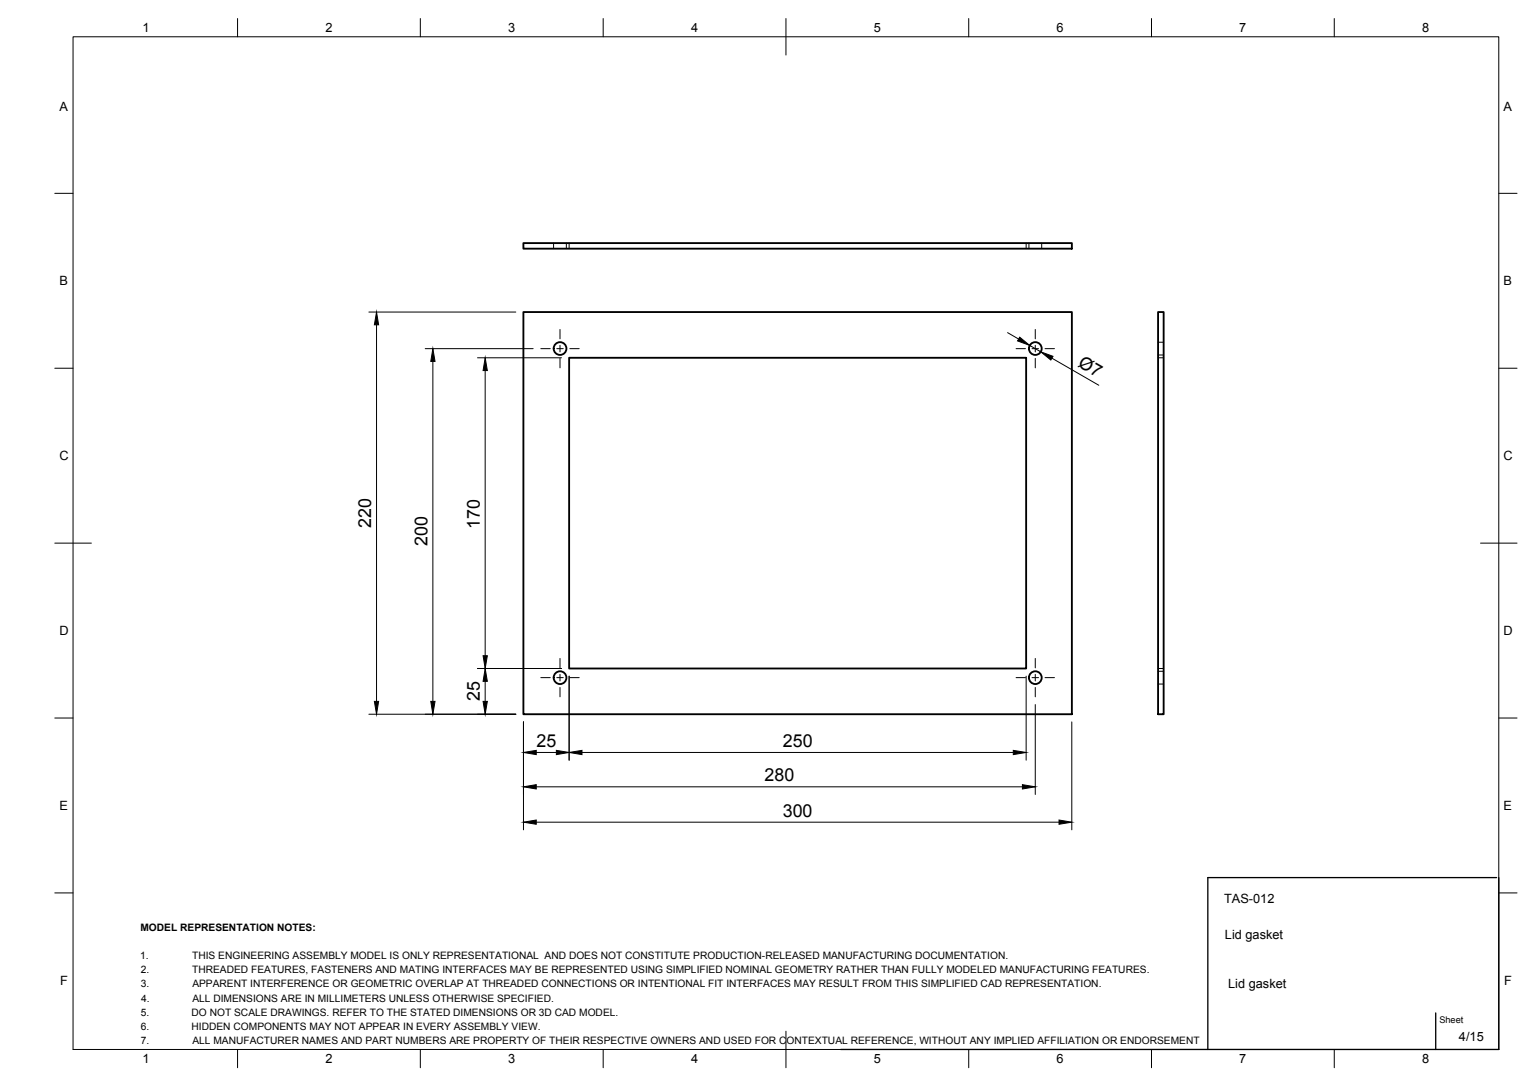
ISO-10303-21;
HEADER;
/* Generated by software containing ST-Developer
 * from STEP Tools, Inc. (www.steptools.com) 
 */

FILE_DESCRIPTION(
/* description */ (
'Independent welded steel electronics enclosure with removable sealed 
lid, internal mounting tray and two threaded cable entries. 300 x 220 
mm body. No ingress or electrical safety rating assigned.'),
/* implementation_level */ '2;1');

FILE_NAME(
/* name */ 'Lid gasket.step',
/* time_stamp */ '2026-11-14T09:13:27-08:00',
/* author */ (''),
/* organization */ (''),
/* preprocessor_version */ 'ST-DEVELOPER v20.2',
/* originating_system */ 'Autodesk Translation Framework v15.17.0.0',
/* authorisation */ '');

FILE_SCHEMA (('AUTOMOTIVE_DESIGN { 1 0 10303 214 3 1 1 }'));
ENDSEC;

DATA;
#10=MECHANICAL_DESIGN_GEOMETRIC_PRESENTATION_REPRESENTATION('',(#974),#94412);
#944=SHAPE_REPRESENTATION_RELATIONSHIP('SRR','None',#94496,#959);
#959=ADVANCED_BREP_SHAPE_REPRESENTATION('',(#989),#94405);
#974=STYLED_ITEM('',(#94578),#989);
#989=MANIFOLD_SOLID_BREP('Body1',#8259);
#1025=FACE_BOUND('',#1770,.T.);
#1026=FACE_BOUND('',#1771,.T.);
#1027=FACE_BOUND('',#1772,.T.);
#1028=FACE_BOUND('',#1773,.T.);
#1029=FACE_BOUND('',#1774,.T.);
#1030=FACE_BOUND('',#1776,.T.);
#1031=FACE_BOUND('',#1777,.T.);
#1032=FACE_BOUND('',#1778,.T.);
#1033=FACE_BOUND('',#1779,.T.);
#1034=FACE_BOUND('',#1780,.T.);
#1115=PLANE('',#8744);
#1116=PLANE('',#8745);
#1117=PLANE('',#8746);
#1118=PLANE('',#8747);
#1119=PLANE('',#8748);
#1120=PLANE('',#8749);
#1121=PLANE('',#8750);
#1122=PLANE('',#8751);
#1123=PLANE('',#8752);
#1124=PLANE('',#8753);
#1372=FACE_OUTER_BOUND('',#1757,.T.);
#1373=FACE_OUTER_BOUND('',#1758,.T.);
#1374=FACE_OUTER_BOUND('',#1759,.T.);
#1375=FACE_OUTER_BOUND('',#1760,.T.);
#1376=FACE_OUTER_BOUND('',#1761,.T.);
#1377=FACE_OUTER_BOUND('',#1762,.T.);
#1378=FACE_OUTER_BOUND('',#1763,.T.);
#1379=FACE_OUTER_BOUND('',#1764,.T.);
#1380=FACE_OUTER_BOUND('',#1765,.T.);
#1381=FACE_OUTER_BOUND('',#1766,.T.);
#1382=FACE_OUTER_BOUND('',#1767,.T.);
#1383=FACE_OUTER_BOUND('',#1768,.T.);
#1384=FACE_OUTER_BOUND('',#1769,.T.);
#1385=FACE_OUTER_BOUND('',#1775,.T.);
#1757=EDGE_LOOP('',(#6692,#6693,#6694,#6695));
#1758=EDGE_LOOP('',(#6696,#6697,#6698,#6699));
#1759=EDGE_LOOP('',(#6700,#6701,#6702,#6703));
#1760=EDGE_LOOP('',(#6704,#6705,#6706,#6707));
#1761=EDGE_LOOP('',(#6708,#6709,#6710,#6711));
#1762=EDGE_LOOP('',(#6712,#6713,#6714,#6715));
#1763=EDGE_LOOP('',(#6716,#6717,#6718,#6719));
#1764=EDGE_LOOP('',(#6720,#6721,#6722,#6723));
#1765=EDGE_LOOP('',(#6724,#6725,#6726,#6727));
#1766=EDGE_LOOP('',(#6728,#6729,#6730,#6731));
#1767=EDGE_LOOP('',(#6732,#6733,#6734,#6735));
#1768=EDGE_LOOP('',(#6736,#6737,#6738,#6739));
#1769=EDGE_LOOP('',(#6740,#6741,#6742,#6743));
#1770=EDGE_LOOP('',(#6744,#6745,#6746,#6747));
#1771=EDGE_LOOP('',(#6748));
#1772=EDGE_LOOP('',(#6749));
#1773=EDGE_LOOP('',(#6750));
#1774=EDGE_LOOP('',(#6751));
#1775=EDGE_LOOP('',(#6752,#6753,#6754,#6755));
#1776=EDGE_LOOP('',(#6756,#6757,#6758,#6759));
#1777=EDGE_LOOP('',(#6760));
#1778=EDGE_LOOP('',(#6761));
#1779=EDGE_LOOP('',(#6762));
#1780=EDGE_LOOP('',(#6763));
#2175=LINE('',#59753,#2573);
#2176=LINE('',#59759,#2574);
#2177=LINE('',#59765,#2575);
#2178=LINE('',#59771,#2576);
#2179=LINE('',#59776,#2577);
#2180=LINE('',#59778,#2578);
#2181=LINE('',#59780,#2579);
#2182=LINE('',#59781,#2580);
#2183=LINE('',#59784,#2581);
#2184=LINE('',#59786,#2582);
#2185=LINE('',#59787,#2583);
#2186=LINE('',#59790,#2584);
#2187=LINE('',#59792,#2585);
#2188=LINE('',#59793,#2586);
#2189=LINE('',#59795,#2587);
#2190=LINE('',#59796,#2588);
#2191=LINE('',#59800,#2589);
#2192=LINE('',#59802,#2590);
#2193=LINE('',#59804,#2591);
#2194=LINE('',#59805,#2592);
#2195=LINE('',#59808,#2593);
#2196=LINE('',#59810,#2594);
#2197=LINE('',#59811,#2595);
#2198=LINE('',#59814,#2596);
#2199=LINE('',#59816,#2597);
#2200=LINE('',#59817,#2598);
#2201=LINE('',#59819,#2599);
#2202=LINE('',#59820,#2600);
#2573=VECTOR('',#9789,3.5);
#2574=VECTOR('',#9796,3.5);
#2575=VECTOR('',#9803,3.5);
#2576=VECTOR('',#9810,3.5);
#2577=VECTOR('',#9815,10.);
#2578=VECTOR('',#9816,10.);
#2579=VECTOR('',#9817,10.);
#2580=VECTOR('',#9818,10.);
#2581=VECTOR('',#9821,10.);
#2582=VECTOR('',#9822,10.);
#2583=VECTOR('',#9823,10.);
#2584=VECTOR('',#9826,10.);
#2585=VECTOR('',#9827,10.);
#2586=VECTOR('',#9828,10.);
#2587=VECTOR('',#9831,10.);
#2588=VECTOR('',#9832,10.);
#2589=VECTOR('',#9835,10.);
#2590=VECTOR('',#9836,10.);
#2591=VECTOR('',#9837,10.);
#2592=VECTOR('',#9838,10.);
#2593=VECTOR('',#9841,10.);
#2594=VECTOR('',#9842,10.);
#2595=VECTOR('',#9843,10.);
#2596=VECTOR('',#9846,10.);
#2597=VECTOR('',#9847,10.);
#2598=VECTOR('',#9848,10.);
#2599=VECTOR('',#9851,10.);
#2600=VECTOR('',#9852,10.);
#2794=CIRCLE('',#8733,3.5);
#2795=CIRCLE('',#8734,3.5);
#2796=CIRCLE('',#8736,3.5);
#2797=CIRCLE('',#8737,3.5);
#2798=CIRCLE('',#8739,3.5);
#2799=CIRCLE('',#8740,3.5);
#2800=CIRCLE('',#8742,3.5);
#2801=CIRCLE('',#8743,3.5);
#3452=VERTEX_POINT('',#59750);
#3453=VERTEX_POINT('',#59752);
#3454=VERTEX_POINT('',#59756);
#3455=VERTEX_POINT('',#59758);
#3456=VERTEX_POINT('',#59762);
#3457=VERTEX_POINT('',#59764);
#3458=VERTEX_POINT('',#59768);
#3459=VERTEX_POINT('',#59770);
#3460=VERTEX_POINT('',#59774);
#3461=VERTEX_POINT('',#59775);
#3462=VERTEX_POINT('',#59777);
#3463=VERTEX_POINT('',#59779);
#3464=VERTEX_POINT('',#59783);
#3465=VERTEX_POINT('',#59785);
#3466=VERTEX_POINT('',#59789);
#3467=VERTEX_POINT('',#59791);
#3468=VERTEX_POINT('',#59798);
#3469=VERTEX_POINT('',#59799);
#3470=VERTEX_POINT('',#59801);
#3471=VERTEX_POINT('',#59803);
#3472=VERTEX_POINT('',#59807);
#3473=VERTEX_POINT('',#59809);
#3474=VERTEX_POINT('',#59813);
#3475=VERTEX_POINT('',#59815);
#4611=EDGE_CURVE('',#3452,#3452,#2794,.T.);
#4612=EDGE_CURVE('',#3452,#3453,#2175,.T.);
#4613=EDGE_CURVE('',#3453,#3453,#2795,.T.);
#4614=EDGE_CURVE('',#3454,#3454,#2796,.T.);
#4615=EDGE_CURVE('',#3454,#3455,#2176,.T.);
#4616=EDGE_CURVE('',#3455,#3455,#2797,.T.);
#4617=EDGE_CURVE('',#3456,#3456,#2798,.T.);
#4618=EDGE_CURVE('',#3456,#3457,#2177,.T.);
#4619=EDGE_CURVE('',#3457,#3457,#2799,.T.);
#4620=EDGE_CURVE('',#3458,#3458,#2800,.T.);
#4621=EDGE_CURVE('',#3458,#3459,#2178,.T.);
#4622=EDGE_CURVE('',#3459,#3459,#2801,.T.);
#4623=EDGE_CURVE('',#3460,#3461,#2179,.T.);
#4624=EDGE_CURVE('',#3461,#3462,#2180,.T.);
#4625=EDGE_CURVE('',#3463,#3462,#2181,.T.);
#4626=EDGE_CURVE('',#3460,#3463,#2182,.T.);
#4627=EDGE_CURVE('',#3464,#3460,#2183,.T.);
#4628=EDGE_CURVE('',#3465,#3463,#2184,.T.);
#4629=EDGE_CURVE('',#3464,#3465,#2185,.T.);
#4630=EDGE_CURVE('',#3466,#3464,#2186,.T.);
#4631=EDGE_CURVE('',#3467,#3465,#2187,.T.);
#4632=EDGE_CURVE('',#3466,#3467,#2188,.T.);
#4633=EDGE_CURVE('',#3461,#3466,#2189,.T.);
#4634=EDGE_CURVE('',#3462,#3467,#2190,.T.);
#4635=EDGE_CURVE('',#3468,#3469,#2191,.T.);
#4636=EDGE_CURVE('',#3469,#3470,#2192,.T.);
#4637=EDGE_CURVE('',#3471,#3470,#2193,.T.);
#4638=EDGE_CURVE('',#3468,#3471,#2194,.T.);
#4639=EDGE_CURVE('',#3472,#3468,#2195,.T.);
#4640=EDGE_CURVE('',#3473,#3471,#2196,.T.);
#4641=EDGE_CURVE('',#3472,#3473,#2197,.T.);
#4642=EDGE_CURVE('',#3474,#3472,#2198,.T.);
#4643=EDGE_CURVE('',#3475,#3473,#2199,.T.);
#4644=EDGE_CURVE('',#3474,#3475,#2200,.T.);
#4645=EDGE_CURVE('',#3469,#3474,#2201,.T.);
#4646=EDGE_CURVE('',#3470,#3475,#2202,.T.);
#6692=ORIENTED_EDGE('',*,*,#4611,.F.);
#6693=ORIENTED_EDGE('',*,*,#4612,.T.);
#6694=ORIENTED_EDGE('',*,*,#4613,.F.);
#6695=ORIENTED_EDGE('',*,*,#4612,.F.);
#6696=ORIENTED_EDGE('',*,*,#4614,.F.);
#6697=ORIENTED_EDGE('',*,*,#4615,.T.);
#6698=ORIENTED_EDGE('',*,*,#4616,.F.);
#6699=ORIENTED_EDGE('',*,*,#4615,.F.);
#6700=ORIENTED_EDGE('',*,*,#4617,.F.);
#6701=ORIENTED_EDGE('',*,*,#4618,.T.);
#6702=ORIENTED_EDGE('',*,*,#4619,.F.);
#6703=ORIENTED_EDGE('',*,*,#4618,.F.);
#6704=ORIENTED_EDGE('',*,*,#4620,.F.);
#6705=ORIENTED_EDGE('',*,*,#4621,.T.);
#6706=ORIENTED_EDGE('',*,*,#4622,.F.);
#6707=ORIENTED_EDGE('',*,*,#4621,.F.);
#6708=ORIENTED_EDGE('',*,*,#4623,.T.);
#6709=ORIENTED_EDGE('',*,*,#4624,.T.);
#6710=ORIENTED_EDGE('',*,*,#4625,.F.);
#6711=ORIENTED_EDGE('',*,*,#4626,.F.);
#6712=ORIENTED_EDGE('',*,*,#4627,.T.);
#6713=ORIENTED_EDGE('',*,*,#4626,.T.);
#6714=ORIENTED_EDGE('',*,*,#4628,.F.);
#6715=ORIENTED_EDGE('',*,*,#4629,.F.);
#6716=ORIENTED_EDGE('',*,*,#4630,.T.);
#6717=ORIENTED_EDGE('',*,*,#4629,.T.);
#6718=ORIENTED_EDGE('',*,*,#4631,.F.);
#6719=ORIENTED_EDGE('',*,*,#4632,.F.);
#6720=ORIENTED_EDGE('',*,*,#4633,.T.);
#6721=ORIENTED_EDGE('',*,*,#4632,.T.);
#6722=ORIENTED_EDGE('',*,*,#4634,.F.);
#6723=ORIENTED_EDGE('',*,*,#4624,.F.);
#6724=ORIENTED_EDGE('',*,*,#4635,.T.);
#6725=ORIENTED_EDGE('',*,*,#4636,.T.);
#6726=ORIENTED_EDGE('',*,*,#4637,.F.);
#6727=ORIENTED_EDGE('',*,*,#4638,.F.);
#6728=ORIENTED_EDGE('',*,*,#4639,.T.);
#6729=ORIENTED_EDGE('',*,*,#4638,.T.);
#6730=ORIENTED_EDGE('',*,*,#4640,.F.);
#6731=ORIENTED_EDGE('',*,*,#4641,.F.);
#6732=ORIENTED_EDGE('',*,*,#4642,.T.);
#6733=ORIENTED_EDGE('',*,*,#4641,.T.);
#6734=ORIENTED_EDGE('',*,*,#4643,.F.);
#6735=ORIENTED_EDGE('',*,*,#4644,.F.);
#6736=ORIENTED_EDGE('',*,*,#4645,.T.);
#6737=ORIENTED_EDGE('',*,*,#4644,.T.);
#6738=ORIENTED_EDGE('',*,*,#4646,.F.);
#6739=ORIENTED_EDGE('',*,*,#4636,.F.);
#6740=ORIENTED_EDGE('',*,*,#4646,.T.);
#6741=ORIENTED_EDGE('',*,*,#4643,.T.);
#6742=ORIENTED_EDGE('',*,*,#4640,.T.);
#6743=ORIENTED_EDGE('',*,*,#4637,.T.);
#6744=ORIENTED_EDGE('',*,*,#4634,.T.);
#6745=ORIENTED_EDGE('',*,*,#4631,.T.);
#6746=ORIENTED_EDGE('',*,*,#4628,.T.);
#6747=ORIENTED_EDGE('',*,*,#4625,.T.);
#6748=ORIENTED_EDGE('',*,*,#4620,.T.);
#6749=ORIENTED_EDGE('',*,*,#4617,.T.);
#6750=ORIENTED_EDGE('',*,*,#4614,.T.);
#6751=ORIENTED_EDGE('',*,*,#4611,.T.);
#6752=ORIENTED_EDGE('',*,*,#4645,.F.);
#6753=ORIENTED_EDGE('',*,*,#4635,.F.);
#6754=ORIENTED_EDGE('',*,*,#4639,.F.);
#6755=ORIENTED_EDGE('',*,*,#4642,.F.);
#6756=ORIENTED_EDGE('',*,*,#4633,.F.);
#6757=ORIENTED_EDGE('',*,*,#4623,.F.);
#6758=ORIENTED_EDGE('',*,*,#4627,.F.);
#6759=ORIENTED_EDGE('',*,*,#4630,.F.);
#6760=ORIENTED_EDGE('',*,*,#4622,.T.);
#6761=ORIENTED_EDGE('',*,*,#4619,.T.);
#6762=ORIENTED_EDGE('',*,*,#4616,.T.);
#6763=ORIENTED_EDGE('',*,*,#4613,.T.);
#7806=CYLINDRICAL_SURFACE('',#8732,3.5);
#7807=CYLINDRICAL_SURFACE('',#8735,3.5);
#7808=CYLINDRICAL_SURFACE('',#8738,3.5);
#7809=CYLINDRICAL_SURFACE('',#8741,3.5);
#8109=ADVANCED_FACE('',(#1372),#7806,.F.);
#8110=ADVANCED_FACE('',(#1373),#7807,.F.);
#8111=ADVANCED_FACE('',(#1374),#7808,.F.);
#8112=ADVANCED_FACE('',(#1375),#7809,.F.);
#8113=ADVANCED_FACE('',(#1376),#1115,.T.);
#8114=ADVANCED_FACE('',(#1377),#1116,.T.);
#8115=ADVANCED_FACE('',(#1378),#1117,.T.);
#8116=ADVANCED_FACE('',(#1379),#1118,.T.);
#8117=ADVANCED_FACE('',(#1380),#1119,.T.);
#8118=ADVANCED_FACE('',(#1381),#1120,.T.);
#8119=ADVANCED_FACE('',(#1382),#1121,.T.);
#8120=ADVANCED_FACE('',(#1383),#1122,.T.);
#8121=ADVANCED_FACE('',(#1384,#1025,#1026,#1027,#1028,#1029),#1123,.T.);
#8122=ADVANCED_FACE('',(#1385,#1030,#1031,#1032,#1033,#1034),#1124,.F.);
#8259=CLOSED_SHELL('',(#8109,#8110,#8111,#8112,#8113,#8114,#8115,#8116,
#8117,#8118,#8119,#8120,#8121,#8122));
#8731=AXIS2_PLACEMENT_3D('',#59748,#9783,#9784);
#8732=AXIS2_PLACEMENT_3D('',#59749,#9785,#9786);
#8733=AXIS2_PLACEMENT_3D('',#59751,#9787,#9788);
#8734=AXIS2_PLACEMENT_3D('',#59754,#9790,#9791);
#8735=AXIS2_PLACEMENT_3D('',#59755,#9792,#9793);
#8736=AXIS2_PLACEMENT_3D('',#59757,#9794,#9795);
#8737=AXIS2_PLACEMENT_3D('',#59760,#9797,#9798);
#8738=AXIS2_PLACEMENT_3D('',#59761,#9799,#9800);
#8739=AXIS2_PLACEMENT_3D('',#59763,#9801,#9802);
#8740=AXIS2_PLACEMENT_3D('',#59766,#9804,#9805);
#8741=AXIS2_PLACEMENT_3D('',#59767,#9806,#9807);
#8742=AXIS2_PLACEMENT_3D('',#59769,#9808,#9809);
#8743=AXIS2_PLACEMENT_3D('',#59772,#9811,#9812);
#8744=AXIS2_PLACEMENT_3D('',#59773,#9813,#9814);
#8745=AXIS2_PLACEMENT_3D('',#59782,#9819,#9820);
#8746=AXIS2_PLACEMENT_3D('',#59788,#9824,#9825);
#8747=AXIS2_PLACEMENT_3D('',#59794,#9829,#9830);
#8748=AXIS2_PLACEMENT_3D('',#59797,#9833,#9834);
#8749=AXIS2_PLACEMENT_3D('',#59806,#9839,#9840);
#8750=AXIS2_PLACEMENT_3D('',#59812,#9844,#9845);
#8751=AXIS2_PLACEMENT_3D('',#59818,#9849,#9850);
#8752=AXIS2_PLACEMENT_3D('',#59821,#9853,#9854);
#8753=AXIS2_PLACEMENT_3D('',#59822,#9855,#9856);
#9783=DIRECTION('axis',(0.,0.,1.));
#9784=DIRECTION('refdir',(1.,0.,0.));
#9785=DIRECTION('center_axis',(0.,0.,-1.));
#9786=DIRECTION('ref_axis',(1.,0.,0.));
#9787=DIRECTION('center_axis',(0.,0.,-1.));
#9788=DIRECTION('ref_axis',(1.,0.,0.));
#9789=DIRECTION('',(0.,0.,-1.));
#9790=DIRECTION('center_axis',(0.,0.,1.));
#9791=DIRECTION('ref_axis',(1.,0.,0.));
#9792=DIRECTION('center_axis',(0.,0.,-1.));
#9793=DIRECTION('ref_axis',(1.,0.,0.));
#9794=DIRECTION('center_axis',(0.,0.,-1.));
#9795=DIRECTION('ref_axis',(1.,0.,0.));
#9796=DIRECTION('',(0.,0.,-1.));
#9797=DIRECTION('center_axis',(0.,0.,1.));
#9798=DIRECTION('ref_axis',(1.,0.,0.));
#9799=DIRECTION('center_axis',(0.,0.,-1.));
#9800=DIRECTION('ref_axis',(1.,0.,0.));
#9801=DIRECTION('center_axis',(0.,0.,-1.));
#9802=DIRECTION('ref_axis',(1.,0.,0.));
#9803=DIRECTION('',(0.,0.,-1.));
#9804=DIRECTION('center_axis',(0.,0.,1.));
#9805=DIRECTION('ref_axis',(1.,0.,0.));
#9806=DIRECTION('center_axis',(0.,0.,-1.));
#9807=DIRECTION('ref_axis',(1.,0.,0.));
#9808=DIRECTION('center_axis',(0.,0.,-1.));
#9809=DIRECTION('ref_axis',(1.,0.,0.));
#9810=DIRECTION('',(0.,0.,-1.));
#9811=DIRECTION('center_axis',(0.,0.,1.));
#9812=DIRECTION('ref_axis',(1.,0.,0.));
#9813=DIRECTION('center_axis',(0.,1.,0.));
#9814=DIRECTION('ref_axis',(-1.,0.,0.));
#9815=DIRECTION('',(-1.,0.,0.));
#9816=DIRECTION('',(0.,0.,1.));
#9817=DIRECTION('',(-1.,0.,0.));
#9818=DIRECTION('',(0.,0.,1.));
#9819=DIRECTION('center_axis',(-1.,0.,0.));
#9820=DIRECTION('ref_axis',(0.,-1.,0.));
#9821=DIRECTION('',(0.,-1.,0.));
#9822=DIRECTION('',(0.,-1.,0.));
#9823=DIRECTION('',(0.,0.,1.));
#9824=DIRECTION('center_axis',(0.,-1.,0.));
#9825=DIRECTION('ref_axis',(1.,0.,0.));
#9826=DIRECTION('',(1.,0.,0.));
#9827=DIRECTION('',(1.,0.,0.));
#9828=DIRECTION('',(0.,0.,1.));
#9829=DIRECTION('center_axis',(1.,0.,0.));
#9830=DIRECTION('ref_axis',(0.,1.,0.));
#9831=DIRECTION('',(0.,1.,0.));
#9832=DIRECTION('',(0.,1.,0.));
#9833=DIRECTION('center_axis',(0.,1.,0.));
#9834=DIRECTION('ref_axis',(-1.,0.,0.));
#9835=DIRECTION('',(-1.,0.,0.));
#9836=DIRECTION('',(0.,0.,1.));
#9837=DIRECTION('',(-1.,0.,0.));
#9838=DIRECTION('',(0.,0.,1.));
#9839=DIRECTION('center_axis',(1.,0.,0.));
#9840=DIRECTION('ref_axis',(0.,1.,0.));
#9841=DIRECTION('',(0.,1.,0.));
#9842=DIRECTION('',(0.,1.,0.));
#9843=DIRECTION('',(0.,0.,1.));
#9844=DIRECTION('center_axis',(0.,-1.,0.));
#9845=DIRECTION('ref_axis',(1.,0.,0.));
#9846=DIRECTION('',(1.,0.,0.));
#9847=DIRECTION('',(1.,0.,0.));
#9848=DIRECTION('',(0.,0.,1.));
#9849=DIRECTION('center_axis',(-1.,0.,0.));
#9850=DIRECTION('ref_axis',(0.,-1.,0.));
#9851=DIRECTION('',(0.,-1.,0.));
#9852=DIRECTION('',(0.,-1.,0.));
#9853=DIRECTION('center_axis',(0.,0.,1.));
#9854=DIRECTION('ref_axis',(1.,0.,0.));
#9855=DIRECTION('center_axis',(0.,0.,1.));
#9856=DIRECTION('ref_axis',(1.,0.,0.));
#59748=CARTESIAN_POINT('',(0.,0.,0.));
#59749=CARTESIAN_POINT('Origin',(130.,-90.,1.5));
#59750=CARTESIAN_POINT('',(126.5,-90.,3.));
#59751=CARTESIAN_POINT('Origin',(130.,-90.,3.));
#59752=CARTESIAN_POINT('',(126.5,-90.,0.));
#59753=CARTESIAN_POINT('',(126.5,-90.,1.5));
#59754=CARTESIAN_POINT('Origin',(130.,-90.,0.));
#59755=CARTESIAN_POINT('Origin',(-130.,-90.,1.5));
#59756=CARTESIAN_POINT('',(-133.5,-90.,3.));
#59757=CARTESIAN_POINT('Origin',(-130.,-90.,3.));
#59758=CARTESIAN_POINT('',(-133.5,-90.,0.));
#59759=CARTESIAN_POINT('',(-133.5,-90.,1.5));
#59760=CARTESIAN_POINT('Origin',(-130.,-90.,0.));
#59761=CARTESIAN_POINT('Origin',(-130.,90.,1.5));
#59762=CARTESIAN_POINT('',(-133.5,90.,3.));
#59763=CARTESIAN_POINT('Origin',(-130.,90.,3.));
#59764=CARTESIAN_POINT('',(-133.5,90.,0.));
#59765=CARTESIAN_POINT('',(-133.5,90.,1.5));
#59766=CARTESIAN_POINT('Origin',(-130.,90.,0.));
#59767=CARTESIAN_POINT('Origin',(130.,90.,1.5));
#59768=CARTESIAN_POINT('',(126.5,90.,3.));
#59769=CARTESIAN_POINT('Origin',(130.,90.,3.));
#59770=CARTESIAN_POINT('',(126.5,90.,0.));
#59771=CARTESIAN_POINT('',(126.5,90.,1.5));
#59772=CARTESIAN_POINT('Origin',(130.,90.,0.));
#59773=CARTESIAN_POINT('Origin',(125.,-85.,0.));
#59774=CARTESIAN_POINT('',(125.,-85.,0.));
#59775=CARTESIAN_POINT('',(-125.,-85.,0.));
#59776=CARTESIAN_POINT('',(-125.,-85.,0.));
#59777=CARTESIAN_POINT('',(-125.,-85.,3.));
#59778=CARTESIAN_POINT('',(-125.,-85.,0.));
#59779=CARTESIAN_POINT('',(125.,-85.,3.));
#59780=CARTESIAN_POINT('',(-125.,-85.,3.));
#59781=CARTESIAN_POINT('',(125.,-85.,0.));
#59782=CARTESIAN_POINT('Origin',(125.,85.,0.));
#59783=CARTESIAN_POINT('',(125.,85.,0.));
#59784=CARTESIAN_POINT('',(125.,-85.,0.));
#59785=CARTESIAN_POINT('',(125.,85.,3.));
#59786=CARTESIAN_POINT('',(125.,-85.,3.));
#59787=CARTESIAN_POINT('',(125.,85.,0.));
#59788=CARTESIAN_POINT('Origin',(-125.,85.,0.));
#59789=CARTESIAN_POINT('',(-125.,85.,0.));
#59790=CARTESIAN_POINT('',(125.,85.,0.));
#59791=CARTESIAN_POINT('',(-125.,85.,3.));
#59792=CARTESIAN_POINT('',(125.,85.,3.));
#59793=CARTESIAN_POINT('',(-125.,85.,0.));
#59794=CARTESIAN_POINT('Origin',(-125.,-85.,0.));
#59795=CARTESIAN_POINT('',(-125.,85.,0.));
#59796=CARTESIAN_POINT('',(-125.,85.,3.));
#59797=CARTESIAN_POINT('Origin',(150.,110.,0.));
#59798=CARTESIAN_POINT('',(150.,110.,0.));
#59799=CARTESIAN_POINT('',(-150.,110.,0.));
#59800=CARTESIAN_POINT('',(150.,110.,0.));
#59801=CARTESIAN_POINT('',(-150.,110.,3.));
#59802=CARTESIAN_POINT('',(-150.,110.,0.));
#59803=CARTESIAN_POINT('',(150.,110.,3.));
#59804=CARTESIAN_POINT('',(150.,110.,3.));
#59805=CARTESIAN_POINT('',(150.,110.,0.));
#59806=CARTESIAN_POINT('Origin',(150.,-110.,0.));
#59807=CARTESIAN_POINT('',(150.,-110.,0.));
#59808=CARTESIAN_POINT('',(150.,-110.,0.));
#59809=CARTESIAN_POINT('',(150.,-110.,3.));
#59810=CARTESIAN_POINT('',(150.,-110.,3.));
#59811=CARTESIAN_POINT('',(150.,-110.,0.));
#59812=CARTESIAN_POINT('Origin',(-150.,-110.,0.));
#59813=CARTESIAN_POINT('',(-150.,-110.,0.));
#59814=CARTESIAN_POINT('',(-150.,-110.,0.));
#59815=CARTESIAN_POINT('',(-150.,-110.,3.));
#59816=CARTESIAN_POINT('',(-150.,-110.,3.));
#59817=CARTESIAN_POINT('',(-150.,-110.,0.));
#59818=CARTESIAN_POINT('Origin',(-150.,110.,0.));
#59819=CARTESIAN_POINT('',(-150.,110.,0.));
#59820=CARTESIAN_POINT('',(-150.,110.,3.));
#59821=CARTESIAN_POINT('Origin',(0.,0.,3.));
#59822=CARTESIAN_POINT('Origin',(0.,0.,0.));
#94387=UNCERTAINTY_MEASURE_WITH_UNIT(LENGTH_MEASURE(0.01),#94413,
'DISTANCE_ACCURACY_VALUE',
'Maximum model space distance between geometric entities at asserted c
onnectivities');
#94394=UNCERTAINTY_MEASURE_WITH_UNIT(LENGTH_MEASURE(0.01),#94413,
'DISTANCE_ACCURACY_VALUE',
'Maximum model space distance between geometric entities at asserted c
onnectivities');
#94405=(
GEOMETRIC_REPRESENTATION_CONTEXT(3)
GLOBAL_UNCERTAINTY_ASSIGNED_CONTEXT((#94387))
GLOBAL_UNIT_ASSIGNED_CONTEXT((#94413,#94415,#94416))
REPRESENTATION_CONTEXT('','3D')
);
#94412=(
GEOMETRIC_REPRESENTATION_CONTEXT(3)
GLOBAL_UNCERTAINTY_ASSIGNED_CONTEXT((#94394))
GLOBAL_UNIT_ASSIGNED_CONTEXT((#94413,#94415,#94416))
REPRESENTATION_CONTEXT('','3D')
);
#94413=(
LENGTH_UNIT()
NAMED_UNIT(*)
SI_UNIT(.MILLI.,.METRE.)
);
#94415=(
NAMED_UNIT(*)
PLANE_ANGLE_UNIT()
SI_UNIT($,.RADIAN.)
);
#94416=(
NAMED_UNIT(*)
SI_UNIT($,.STERADIAN.)
SOLID_ANGLE_UNIT()
);
#94427=SHAPE_DEFINITION_REPRESENTATION(#94461,#94496);
#94461=PRODUCT_DEFINITION_SHAPE('',$,#94514);
#94496=SHAPE_REPRESENTATION('',(#8731),#94405);
#94503=PRODUCT_DEFINITION_CONTEXT('part definition',#94556,'design');
#94514=PRODUCT_DEFINITION('Lid gasket','Lid gasket',#94531,#94503);
#94531=PRODUCT_DEFINITION_FORMATION('',$,#94568);
#94556=APPLICATION_CONTEXT(
'Core Data for Automotive Mechanical Design Process');
#94557=PRODUCT_CONTEXT('part definition',#94556,'mechanical');
#94568=PRODUCT('Lid gasket','Lid gasket',
'Closed-cell elastomer gasket, nominal 3 mm thickness. Seal compressio
n and environmental rating require validation.',(#94557));
#94578=PRESENTATION_STYLE_ASSIGNMENT((#94585));
#94585=SURFACE_STYLE_USAGE(.BOTH.,#94592);
#94592=SURFACE_SIDE_STYLE('',(#94599));
#94599=SURFACE_STYLE_FILL_AREA(#94606);
#94606=FILL_AREA_STYLE('Opaque(64,72,82)',(#94613));
#94613=FILL_AREA_STYLE_COLOUR('Opaque(64,72,82)',#94620);
#94620=COLOUR_RGB('Opaque(64,72,82)',0.250980392156863,0.282352941176471,
0.32156862745098);
ENDSEC;
END-ISO-10303-21;
